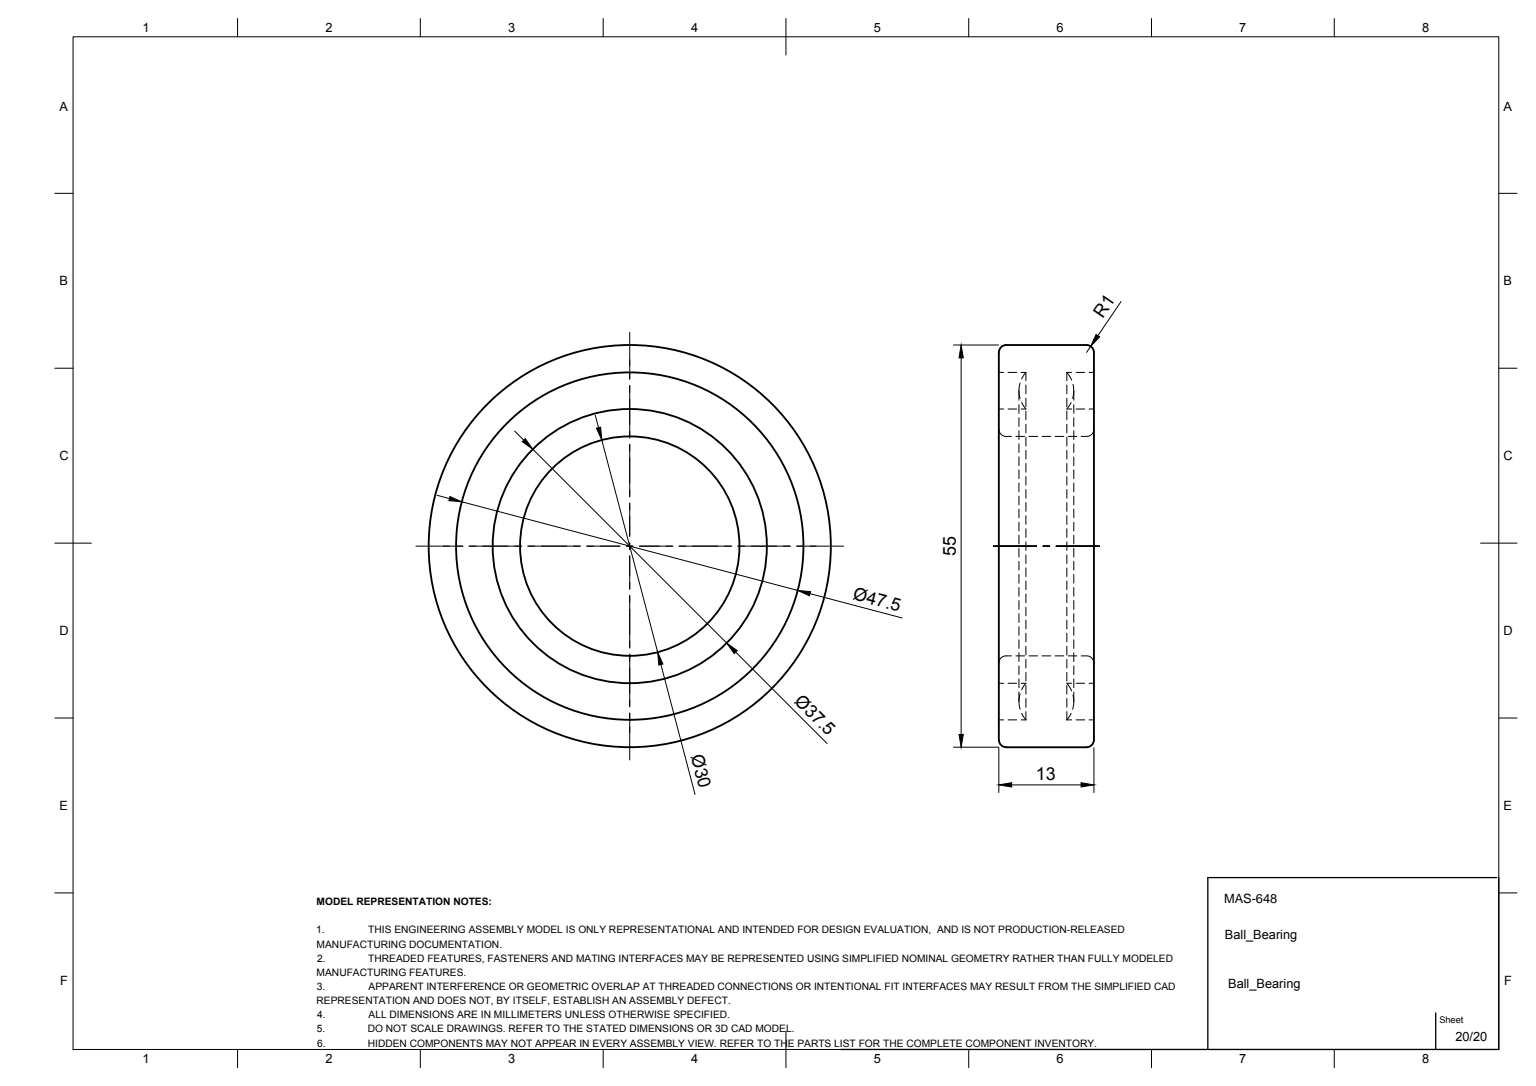
ISO-10303-21;
HEADER;
FILE_DESCRIPTION((''),'2;1');
FILE_NAME('Ball_Bearing.step','2026-10-09T12:47:58-07:00',(''),(''),'','','');
FILE_SCHEMA (('AUTOMOTIVE_DESIGN { 1 0 10303 214 3 1 1 }'));
ENDSEC;
DATA;
#10=MECHANICAL_DESIGN_GEOMETRIC_PRESENTATION_REPRESENTATION('',(#320),#3475);
#24=TOROIDAL_SURFACE('',#2119,26.5,1.) ;
#25=TOROIDAL_SURFACE('',#2125,26.5,1.) ;
#26=TOROIDAL_SURFACE('',#2136,21.25,3.75) ;
#27=TOROIDAL_SURFACE('',#2140,16.,1.) ;
#28=TOROIDAL_SURFACE('',#2146,16.,1.) ;
#29=TOROIDAL_SURFACE('',#2155,21.25,3.75) ;
#161=FACE_BOUND('',#554,.T.) ;
#162=FACE_BOUND('',#556,.T.) ;
#163=FACE_BOUND('',#558,.T.) ;
#164=FACE_BOUND('',#560,.T.) ;
#211=CIRCLE('',#2120,27.5) ;
#212=CIRCLE('',#2121,1.) ;
#213=CIRCLE('',#2122,26.5) ;
#214=CIRCLE('',#2124,27.5) ;
#215=CIRCLE('',#2126,26.5) ;
#216=CIRCLE('',#2127,1.) ;
#217=CIRCLE('',#2129,23.75) ;
#218=CIRCLE('',#2130,23.75) ;
#219=CIRCLE('',#2131,23.75) ;
#220=CIRCLE('',#2133,23.75) ;
#221=CIRCLE('',#2134,23.75) ;
#222=CIRCLE('',#2135,23.75) ;
#223=CIRCLE('',#2137,18.75) ;
#224=CIRCLE('',#2138,3.75) ;
#225=CIRCLE('',#2139,18.75) ;
#226=CIRCLE('',#2141,16.) ;
#227=CIRCLE('',#2142,1.) ;
#228=CIRCLE('',#2143,15.) ;
#229=CIRCLE('',#2145,15.) ;
#230=CIRCLE('',#2147,1.) ;
#231=CIRCLE('',#2148,16.) ;
#232=CIRCLE('',#2150,18.75) ;
#233=CIRCLE('',#2152,18.75) ;
#234=CIRCLE('',#2153,18.75) ;
#235=CIRCLE('',#2154,18.75) ;
#236=CIRCLE('',#2156,3.75) ;
#278=CYLINDRICAL_SURFACE('',#2123,27.5) ;
#279=CYLINDRICAL_SURFACE('',#2128,23.75) ;
#280=CYLINDRICAL_SURFACE('',#2132,23.75) ;
#281=CYLINDRICAL_SURFACE('',#2144,15.) ;
#282=CYLINDRICAL_SURFACE('',#2149,18.75) ;
#283=CYLINDRICAL_SURFACE('',#2151,18.75) ;
#296=SHAPE_REPRESENTATION_RELATIONSHIP('SRR','None',#3553,#308) ;
#308=ADVANCED_BREP_SHAPE_REPRESENTATION('',(#332),#3473) ;
#320=STYLED_ITEM('',(#3628),#332) ;
#332=MANIFOLD_SOLID_BREP('Body1',#1834) ;
#407=FACE_OUTER_BOUND('',#541,.T.) ;
#408=FACE_OUTER_BOUND('',#542,.T.) ;
#409=FACE_OUTER_BOUND('',#543,.T.) ;
#410=FACE_OUTER_BOUND('',#544,.T.) ;
#411=FACE_OUTER_BOUND('',#545,.T.) ;
#412=FACE_OUTER_BOUND('',#546,.T.) ;
#413=FACE_OUTER_BOUND('',#547,.T.) ;
#414=FACE_OUTER_BOUND('',#548,.T.) ;
#415=FACE_OUTER_BOUND('',#549,.T.) ;
#416=FACE_OUTER_BOUND('',#550,.T.) ;
#417=FACE_OUTER_BOUND('',#551,.T.) ;
#418=FACE_OUTER_BOUND('',#552,.T.) ;
#419=FACE_OUTER_BOUND('',#553,.T.) ;
#420=FACE_OUTER_BOUND('',#555,.T.) ;
#421=FACE_OUTER_BOUND('',#557,.T.) ;
#422=FACE_OUTER_BOUND('',#559,.T.) ;
#541=EDGE_LOOP('',(#1476,#1477,#1478,#1479)) ;
#542=EDGE_LOOP('',(#1480,#1481,#1482,#1483)) ;
#543=EDGE_LOOP('',(#1484,#1485,#1486,#1487)) ;
#544=EDGE_LOOP('',(#1488,#1489,#1490,#1491,#1492)) ;
#545=EDGE_LOOP('',(#1493,#1494,#1495,#1496,#1497)) ;
#546=EDGE_LOOP('',(#1498,#1499,#1500,#1501,#1502,#1503)) ;
#547=EDGE_LOOP('',(#1504,#1505,#1506,#1507)) ;
#548=EDGE_LOOP('',(#1508,#1509,#1510,#1511)) ;
#549=EDGE_LOOP('',(#1512,#1513,#1514,#1515)) ;
#550=EDGE_LOOP('',(#1516,#1517,#1518,#1519,#1520)) ;
#551=EDGE_LOOP('',(#1521,#1522,#1523,#1524,#1525)) ;
#552=EDGE_LOOP('',(#1526,#1527,#1528,#1529,#1530,#1531)) ;
#553=EDGE_LOOP('',(#1532)) ;
#554=EDGE_LOOP('',(#1533)) ;
#555=EDGE_LOOP('',(#1534)) ;
#556=EDGE_LOOP('',(#1535)) ;
#557=EDGE_LOOP('',(#1536)) ;
#558=EDGE_LOOP('',(#1537)) ;
#559=EDGE_LOOP('',(#1538)) ;
#560=EDGE_LOOP('',(#1539)) ;
#679=LINE('',#3241,#798) ;
#680=LINE('',#3250,#799) ;
#681=LINE('',#3260,#800) ;
#682=LINE('',#3276,#801) ;
#683=LINE('',#3284,#802) ;
#684=LINE('',#3290,#803) ;
#798=VECTOR('',#2618,27.5) ;
#799=VECTOR('',#2629,23.75) ;
#800=VECTOR('',#2640,23.75) ;
#801=VECTOR('',#2661,15.) ;
#802=VECTOR('',#2672,18.75) ;
#803=VECTOR('',#2679,18.75) ;
#919=VERTEX_POINT('',#3233) ;
#920=VERTEX_POINT('',#3235) ;
#921=VERTEX_POINT('',#3239) ;
#922=VERTEX_POINT('',#3243) ;
#923=VERTEX_POINT('',#3247) ;
#924=VERTEX_POINT('',#3249) ;
#925=VERTEX_POINT('',#3251) ;
#926=VERTEX_POINT('',#3255) ;
#927=VERTEX_POINT('',#3256) ;
#928=VERTEX_POINT('',#3259) ;
#929=VERTEX_POINT('',#3263) ;
#930=VERTEX_POINT('',#3264) ;
#931=VERTEX_POINT('',#3269) ;
#932=VERTEX_POINT('',#3271) ;
#933=VERTEX_POINT('',#3275) ;
#934=VERTEX_POINT('',#3279) ;
#935=VERTEX_POINT('',#3283) ;
#936=VERTEX_POINT('',#3287) ;
#937=VERTEX_POINT('',#3289) ;
#938=VERTEX_POINT('',#3291) ;
#1110=EDGE_CURVE('',#919,#919,#211,.T.) ;
#1111=EDGE_CURVE('',#919,#920,#212,.T.) ;
#1112=EDGE_CURVE('',#920,#920,#213,.T.) ;
#1113=EDGE_CURVE('',#921,#921,#214,.T.) ;
#1114=EDGE_CURVE('',#921,#919,#679,.T.) ;
#1115=EDGE_CURVE('',#922,#922,#215,.T.) ;
#1116=EDGE_CURVE('',#922,#921,#216,.T.) ;
#1117=EDGE_CURVE('',#923,#923,#217,.T.) ;
#1118=EDGE_CURVE('',#923,#924,#680,.T.) ;
#1119=EDGE_CURVE('',#925,#924,#218,.T.) ;
#1120=EDGE_CURVE('',#924,#925,#219,.T.) ;
#1121=EDGE_CURVE('',#926,#927,#220,.T.) ;
#1122=EDGE_CURVE('',#927,#926,#221,.T.) ;
#1123=EDGE_CURVE('',#927,#928,#681,.T.) ;
#1124=EDGE_CURVE('',#928,#928,#222,.T.) ;
#1125=EDGE_CURVE('',#929,#930,#223,.T.) ;
#1126=EDGE_CURVE('',#930,#925,#224,.T.) ;
#1127=EDGE_CURVE('',#930,#929,#225,.T.) ;
#1128=EDGE_CURVE('',#931,#931,#226,.T.) ;
#1129=EDGE_CURVE('',#931,#932,#227,.T.) ;
#1130=EDGE_CURVE('',#932,#932,#228,.T.) ;
#1131=EDGE_CURVE('',#932,#933,#682,.T.) ;
#1132=EDGE_CURVE('',#933,#933,#229,.T.) ;
#1133=EDGE_CURVE('',#933,#934,#230,.T.) ;
#1134=EDGE_CURVE('',#934,#934,#231,.T.) ;
#1135=EDGE_CURVE('',#929,#935,#683,.T.) ;
#1136=EDGE_CURVE('',#935,#935,#232,.T.) ;
#1137=EDGE_CURVE('',#936,#936,#233,.T.) ;
#1138=EDGE_CURVE('',#936,#937,#684,.T.) ;
#1139=EDGE_CURVE('',#938,#937,#234,.T.) ;
#1140=EDGE_CURVE('',#937,#938,#235,.T.) ;
#1141=EDGE_CURVE('',#926,#938,#236,.T.) ;
#1476=ORIENTED_EDGE('',*,*,#1110,.F.) ;
#1477=ORIENTED_EDGE('',*,*,#1111,.T.) ;
#1478=ORIENTED_EDGE('',*,*,#1112,.T.) ;
#1479=ORIENTED_EDGE('',*,*,#1111,.F.) ;
#1480=ORIENTED_EDGE('',*,*,#1113,.F.) ;
#1481=ORIENTED_EDGE('',*,*,#1114,.T.) ;
#1482=ORIENTED_EDGE('',*,*,#1110,.T.) ;
#1483=ORIENTED_EDGE('',*,*,#1114,.F.) ;
#1484=ORIENTED_EDGE('',*,*,#1115,.F.) ;
#1485=ORIENTED_EDGE('',*,*,#1116,.T.) ;
#1486=ORIENTED_EDGE('',*,*,#1113,.T.) ;
#1487=ORIENTED_EDGE('',*,*,#1116,.F.) ;
#1488=ORIENTED_EDGE('',*,*,#1117,.F.) ;
#1489=ORIENTED_EDGE('',*,*,#1118,.T.) ;
#1490=ORIENTED_EDGE('',*,*,#1119,.F.) ;
#1491=ORIENTED_EDGE('',*,*,#1120,.F.) ;
#1492=ORIENTED_EDGE('',*,*,#1118,.F.) ;
#1493=ORIENTED_EDGE('',*,*,#1121,.F.) ;
#1494=ORIENTED_EDGE('',*,*,#1122,.F.) ;
#1495=ORIENTED_EDGE('',*,*,#1123,.T.) ;
#1496=ORIENTED_EDGE('',*,*,#1124,.T.) ;
#1497=ORIENTED_EDGE('',*,*,#1123,.F.) ;
#1498=ORIENTED_EDGE('',*,*,#1125,.T.) ;
#1499=ORIENTED_EDGE('',*,*,#1126,.T.) ;
#1500=ORIENTED_EDGE('',*,*,#1119,.T.) ;
#1501=ORIENTED_EDGE('',*,*,#1120,.T.) ;
#1502=ORIENTED_EDGE('',*,*,#1126,.F.) ;
#1503=ORIENTED_EDGE('',*,*,#1127,.T.) ;
#1504=ORIENTED_EDGE('',*,*,#1128,.F.) ;
#1505=ORIENTED_EDGE('',*,*,#1129,.T.) ;
#1506=ORIENTED_EDGE('',*,*,#1130,.T.) ;
#1507=ORIENTED_EDGE('',*,*,#1129,.F.) ;
#1508=ORIENTED_EDGE('',*,*,#1130,.F.) ;
#1509=ORIENTED_EDGE('',*,*,#1131,.T.) ;
#1510=ORIENTED_EDGE('',*,*,#1132,.T.) ;
#1511=ORIENTED_EDGE('',*,*,#1131,.F.) ;
#1512=ORIENTED_EDGE('',*,*,#1132,.F.) ;
#1513=ORIENTED_EDGE('',*,*,#1133,.T.) ;
#1514=ORIENTED_EDGE('',*,*,#1134,.T.) ;
#1515=ORIENTED_EDGE('',*,*,#1133,.F.) ;
#1516=ORIENTED_EDGE('',*,*,#1125,.F.) ;
#1517=ORIENTED_EDGE('',*,*,#1135,.T.) ;
#1518=ORIENTED_EDGE('',*,*,#1136,.T.) ;
#1519=ORIENTED_EDGE('',*,*,#1135,.F.) ;
#1520=ORIENTED_EDGE('',*,*,#1127,.F.) ;
#1521=ORIENTED_EDGE('',*,*,#1137,.F.) ;
#1522=ORIENTED_EDGE('',*,*,#1138,.T.) ;
#1523=ORIENTED_EDGE('',*,*,#1139,.F.) ;
#1524=ORIENTED_EDGE('',*,*,#1140,.F.) ;
#1525=ORIENTED_EDGE('',*,*,#1138,.F.) ;
#1526=ORIENTED_EDGE('',*,*,#1121,.T.) ;
#1527=ORIENTED_EDGE('',*,*,#1122,.T.) ;
#1528=ORIENTED_EDGE('',*,*,#1141,.T.) ;
#1529=ORIENTED_EDGE('',*,*,#1139,.T.) ;
#1530=ORIENTED_EDGE('',*,*,#1140,.T.) ;
#1531=ORIENTED_EDGE('',*,*,#1141,.F.) ;
#1532=ORIENTED_EDGE('',*,*,#1137,.T.) ;
#1533=ORIENTED_EDGE('',*,*,#1134,.F.) ;
#1534=ORIENTED_EDGE('',*,*,#1136,.F.) ;
#1535=ORIENTED_EDGE('',*,*,#1128,.T.) ;
#1536=ORIENTED_EDGE('',*,*,#1115,.T.) ;
#1537=ORIENTED_EDGE('',*,*,#1124,.F.) ;
#1538=ORIENTED_EDGE('',*,*,#1112,.F.) ;
#1539=ORIENTED_EDGE('',*,*,#1117,.T.) ;
#1691=PLANE('',#2157) ;
#1692=PLANE('',#2158) ;
#1693=PLANE('',#2159) ;
#1694=PLANE('',#2160) ;
#1783=ADVANCED_FACE('',(#407),#24,.T.) ;
#1784=ADVANCED_FACE('',(#408),#278,.T.) ;
#1785=ADVANCED_FACE('',(#409),#25,.T.) ;
#1786=ADVANCED_FACE('',(#410),#279,.F.) ;
#1787=ADVANCED_FACE('',(#411),#280,.F.) ;
#1788=ADVANCED_FACE('',(#412),#26,.T.) ;
#1789=ADVANCED_FACE('',(#413),#27,.T.) ;
#1790=ADVANCED_FACE('',(#414),#281,.F.) ;
#1791=ADVANCED_FACE('',(#415),#28,.T.) ;
#1792=ADVANCED_FACE('',(#416),#282,.T.) ;
#1793=ADVANCED_FACE('',(#417),#283,.T.) ;
#1794=ADVANCED_FACE('',(#418),#29,.T.) ;
#1795=ADVANCED_FACE('',(#419,#161),#1691,.T.) ;
#1796=ADVANCED_FACE('',(#420,#162),#1692,.T.) ;
#1797=ADVANCED_FACE('',(#421,#163),#1693,.T.) ;
#1798=ADVANCED_FACE('',(#422,#164),#1694,.T.) ;
#1834=CLOSED_SHELL('',(#1783,#1784,#1785,#1786,#1787,#1788,#1789,#1790,
#1791,#1792,#1793,#1794,#1795,#1796,#1797,#1798)) ;
#2118=AXIS2_PLACEMENT_3D('',#3231,#2604,#2605) ;
#2119=AXIS2_PLACEMENT_3D('',#3232,#2606,#2607) ;
#2120=AXIS2_PLACEMENT_3D('',#3234,#2608,#2609) ;
#2121=AXIS2_PLACEMENT_3D('',#3236,#2610,#2611) ;
#2122=AXIS2_PLACEMENT_3D('',#3237,#2612,#2613) ;
#2123=AXIS2_PLACEMENT_3D('',#3238,#2614,#2615) ;
#2124=AXIS2_PLACEMENT_3D('',#3240,#2616,#2617) ;
#2125=AXIS2_PLACEMENT_3D('',#3242,#2619,#2620) ;
#2126=AXIS2_PLACEMENT_3D('',#3244,#2621,#2622) ;
#2127=AXIS2_PLACEMENT_3D('',#3245,#2623,#2624) ;
#2128=AXIS2_PLACEMENT_3D('',#3246,#2625,#2626) ;
#2129=AXIS2_PLACEMENT_3D('',#3248,#2627,#2628) ;
#2130=AXIS2_PLACEMENT_3D('',#3252,#2630,#2631) ;
#2131=AXIS2_PLACEMENT_3D('',#3253,#2632,#2633) ;
#2132=AXIS2_PLACEMENT_3D('',#3254,#2634,#2635) ;
#2133=AXIS2_PLACEMENT_3D('',#3257,#2636,#2637) ;
#2134=AXIS2_PLACEMENT_3D('',#3258,#2638,#2639) ;
#2135=AXIS2_PLACEMENT_3D('',#3261,#2641,#2642) ;
#2136=AXIS2_PLACEMENT_3D('',#3262,#2643,#2644) ;
#2137=AXIS2_PLACEMENT_3D('',#3265,#2645,#2646) ;
#2138=AXIS2_PLACEMENT_3D('',#3266,#2647,#2648) ;
#2139=AXIS2_PLACEMENT_3D('',#3267,#2649,#2650) ;
#2140=AXIS2_PLACEMENT_3D('',#3268,#2651,#2652) ;
#2141=AXIS2_PLACEMENT_3D('',#3270,#2653,#2654) ;
#2142=AXIS2_PLACEMENT_3D('',#3272,#2655,#2656) ;
#2143=AXIS2_PLACEMENT_3D('',#3273,#2657,#2658) ;
#2144=AXIS2_PLACEMENT_3D('',#3274,#2659,#2660) ;
#2145=AXIS2_PLACEMENT_3D('',#3277,#2662,#2663) ;
#2146=AXIS2_PLACEMENT_3D('',#3278,#2664,#2665) ;
#2147=AXIS2_PLACEMENT_3D('',#3280,#2666,#2667) ;
#2148=AXIS2_PLACEMENT_3D('',#3281,#2668,#2669) ;
#2149=AXIS2_PLACEMENT_3D('',#3282,#2670,#2671) ;
#2150=AXIS2_PLACEMENT_3D('',#3285,#2673,#2674) ;
#2151=AXIS2_PLACEMENT_3D('',#3286,#2675,#2676) ;
#2152=AXIS2_PLACEMENT_3D('',#3288,#2677,#2678) ;
#2153=AXIS2_PLACEMENT_3D('',#3292,#2680,#2681) ;
#2154=AXIS2_PLACEMENT_3D('',#3293,#2682,#2683) ;
#2155=AXIS2_PLACEMENT_3D('',#3294,#2684,#2685) ;
#2156=AXIS2_PLACEMENT_3D('',#3295,#2686,#2687) ;
#2157=AXIS2_PLACEMENT_3D('',#3296,#2688,#2689) ;
#2158=AXIS2_PLACEMENT_3D('',#3297,#2690,#2691) ;
#2159=AXIS2_PLACEMENT_3D('',#3298,#2692,#2693) ;
#2160=AXIS2_PLACEMENT_3D('',#3299,#2694,#2695) ;
#2604=DIRECTION('axis',(0.,0.,1.)) ;
#2605=DIRECTION('refdir',(1.,0.,0.)) ;
#2606=DIRECTION('center_axis',(1.,0.,0.)) ;
#2607=DIRECTION('ref_axis',(0.,0.,-1.)) ;
#2608=DIRECTION('center_axis',(1.,0.,0.)) ;
#2609=DIRECTION('ref_axis',(0.,0.,-1.)) ;
#2610=DIRECTION('center_axis',(0.,-1.,-1.22464679914735E-16)) ;
#2611=DIRECTION('ref_axis',(0.,-1.22464679914735E-16,1.)) ;
#2612=DIRECTION('center_axis',(1.,0.,0.)) ;
#2613=DIRECTION('ref_axis',(0.,0.,-1.)) ;
#2614=DIRECTION('center_axis',(1.,0.,0.)) ;
#2615=DIRECTION('ref_axis',(0.,0.,-1.)) ;
#2616=DIRECTION('center_axis',(1.,0.,0.)) ;
#2617=DIRECTION('ref_axis',(0.,0.,-1.)) ;
#2618=DIRECTION('',(-1.,0.,0.)) ;
#2619=DIRECTION('center_axis',(1.,0.,0.)) ;
#2620=DIRECTION('ref_axis',(0.,0.,-1.)) ;
#2621=DIRECTION('center_axis',(1.,0.,0.)) ;
#2622=DIRECTION('ref_axis',(0.,0.,-1.)) ;
#2623=DIRECTION('center_axis',(0.,-1.,-1.22464679914735E-16)) ;
#2624=DIRECTION('ref_axis',(0.,-1.22464679914735E-16,1.)) ;
#2625=DIRECTION('center_axis',(1.,0.,0.)) ;
#2626=DIRECTION('ref_axis',(0.,0.,-1.)) ;
#2627=DIRECTION('center_axis',(1.,0.,0.)) ;
#2628=DIRECTION('ref_axis',(0.,0.,-1.)) ;
#2629=DIRECTION('',(1.,0.,0.)) ;
#2630=DIRECTION('center_axis',(-1.,0.,0.)) ;
#2631=DIRECTION('ref_axis',(0.,0.,-1.)) ;
#2632=DIRECTION('center_axis',(-1.,0.,0.)) ;
#2633=DIRECTION('ref_axis',(0.,0.,-1.)) ;
#2634=DIRECTION('center_axis',(1.,0.,0.)) ;
#2635=DIRECTION('ref_axis',(0.,0.,-1.)) ;
#2636=DIRECTION('center_axis',(1.,0.,0.)) ;
#2637=DIRECTION('ref_axis',(0.,0.,1.)) ;
#2638=DIRECTION('center_axis',(1.,0.,0.)) ;
#2639=DIRECTION('ref_axis',(0.,0.,1.)) ;
#2640=DIRECTION('',(1.,0.,0.)) ;
#2641=DIRECTION('center_axis',(1.,0.,0.)) ;
#2642=DIRECTION('ref_axis',(0.,0.,-1.)) ;
#2643=DIRECTION('center_axis',(-1.,0.,0.)) ;
#2644=DIRECTION('ref_axis',(0.,0.,1.)) ;
#2645=DIRECTION('center_axis',(1.,0.,0.)) ;
#2646=DIRECTION('ref_axis',(0.,0.,-1.)) ;
#2647=DIRECTION('center_axis',(0.,-1.,1.22464679914735E-16)) ;
#2648=DIRECTION('ref_axis',(0.,-1.22464679914735E-16,-1.)) ;
#2649=DIRECTION('center_axis',(1.,0.,0.)) ;
#2650=DIRECTION('ref_axis',(0.,0.,-1.)) ;
#2651=DIRECTION('center_axis',(1.,0.,0.)) ;
#2652=DIRECTION('ref_axis',(0.,0.,-1.)) ;
#2653=DIRECTION('center_axis',(1.,0.,0.)) ;
#2654=DIRECTION('ref_axis',(0.,0.,-1.)) ;
#2655=DIRECTION('center_axis',(0.,-1.,-1.22464679914735E-16)) ;
#2656=DIRECTION('ref_axis',(0.,-1.22464679914735E-16,1.)) ;
#2657=DIRECTION('center_axis',(1.,0.,0.)) ;
#2658=DIRECTION('ref_axis',(0.,0.,-1.)) ;
#2659=DIRECTION('center_axis',(1.,0.,0.)) ;
#2660=DIRECTION('ref_axis',(0.,0.,-1.)) ;
#2661=DIRECTION('',(1.,0.,0.)) ;
#2662=DIRECTION('center_axis',(1.,0.,0.)) ;
#2663=DIRECTION('ref_axis',(0.,0.,-1.)) ;
#2664=DIRECTION('center_axis',(1.,0.,0.)) ;
#2665=DIRECTION('ref_axis',(0.,0.,-1.)) ;
#2666=DIRECTION('center_axis',(0.,-1.,-1.22464679914735E-16)) ;
#2667=DIRECTION('ref_axis',(0.,-1.22464679914735E-16,1.)) ;
#2668=DIRECTION('center_axis',(1.,0.,0.)) ;
#2669=DIRECTION('ref_axis',(0.,0.,-1.)) ;
#2670=DIRECTION('center_axis',(1.,0.,0.)) ;
#2671=DIRECTION('ref_axis',(0.,0.,-1.)) ;
#2672=DIRECTION('',(-1.,0.,0.)) ;
#2673=DIRECTION('center_axis',(1.,0.,0.)) ;
#2674=DIRECTION('ref_axis',(0.,0.,-1.)) ;
#2675=DIRECTION('center_axis',(1.,0.,0.)) ;
#2676=DIRECTION('ref_axis',(0.,0.,-1.)) ;
#2677=DIRECTION('center_axis',(1.,0.,0.)) ;
#2678=DIRECTION('ref_axis',(0.,0.,-1.)) ;
#2679=DIRECTION('',(-1.,0.,0.)) ;
#2680=DIRECTION('center_axis',(-1.,0.,0.)) ;
#2681=DIRECTION('ref_axis',(0.,0.,1.)) ;
#2682=DIRECTION('center_axis',(-1.,0.,0.)) ;
#2683=DIRECTION('ref_axis',(0.,0.,1.)) ;
#2684=DIRECTION('center_axis',(-1.,0.,0.)) ;
#2685=DIRECTION('ref_axis',(0.,0.,1.)) ;
#2686=DIRECTION('center_axis',(0.,-1.,1.22464679914735E-16)) ;
#2687=DIRECTION('ref_axis',(0.,-1.22464679914735E-16,-1.)) ;
#2688=DIRECTION('center_axis',(1.,0.,0.)) ;
#2689=DIRECTION('ref_axis',(0.,0.,-1.)) ;
#2690=DIRECTION('center_axis',(-1.,0.,0.)) ;
#2691=DIRECTION('ref_axis',(0.,0.,1.)) ;
#2692=DIRECTION('center_axis',(1.,0.,0.)) ;
#2693=DIRECTION('ref_axis',(0.,0.,-1.)) ;
#2694=DIRECTION('center_axis',(-1.,0.,0.)) ;
#2695=DIRECTION('ref_axis',(0.,0.,1.)) ;
#3231=CARTESIAN_POINT('',(0.,0.,0.)) ;
#3232=CARTESIAN_POINT('Origin',(-5.5,0.,0.)) ;
#3233=CARTESIAN_POINT('',(-5.5,-3.36777869765522E-15,27.5)) ;
#3234=CARTESIAN_POINT('Origin',(-5.5,0.,0.)) ;
#3235=CARTESIAN_POINT('',(-6.5,-3.24531401774049E-15,26.5)) ;
#3236=CARTESIAN_POINT('Origin',(-5.5,-3.24531401774049E-15,26.5)) ;
#3237=CARTESIAN_POINT('Origin',(-6.5,0.,0.)) ;
#3238=CARTESIAN_POINT('Origin',(-20.6375,0.,0.)) ;
#3239=CARTESIAN_POINT('',(5.5,-3.36777869765522E-15,27.5)) ;
#3240=CARTESIAN_POINT('Origin',(5.5,0.,0.)) ;
#3241=CARTESIAN_POINT('',(-20.6375,-3.36777869765522E-15,27.5)) ;
#3242=CARTESIAN_POINT('Origin',(5.5,0.,0.)) ;
#3243=CARTESIAN_POINT('',(6.5,-3.24531401774049E-15,26.5)) ;
#3244=CARTESIAN_POINT('Origin',(6.5,0.,0.)) ;
#3245=CARTESIAN_POINT('Origin',(5.5,-3.24531401774049E-15,26.5)) ;
#3246=CARTESIAN_POINT('Origin',(-20.6375,0.,0.)) ;
#3247=CARTESIAN_POINT('',(-6.5,-2.90853614797497E-15,23.75)) ;
#3248=CARTESIAN_POINT('Origin',(-6.5,0.,0.)) ;
#3249=CARTESIAN_POINT('',(-2.79508497187473,-2.90853614797496E-15,23.75)) ;
#3250=CARTESIAN_POINT('',(-20.6375,-2.90853614797496E-15,23.75)) ;
#3251=CARTESIAN_POINT('',(-2.79508497187473,2.90853614797496E-15,-23.75)) ;
#3252=CARTESIAN_POINT('Origin',(-2.79508497187473,0.,0.)) ;
#3253=CARTESIAN_POINT('Origin',(-2.79508497187473,0.,0.)) ;
#3254=CARTESIAN_POINT('Origin',(-20.6375,0.,0.)) ;
#3255=CARTESIAN_POINT('',(2.79508497187473,2.90853614797496E-15,-23.75)) ;
#3256=CARTESIAN_POINT('',(2.79508497187473,-2.90853614797496E-15,23.75)) ;
#3257=CARTESIAN_POINT('Origin',(2.79508497187473,0.,0.)) ;
#3258=CARTESIAN_POINT('Origin',(2.79508497187473,0.,0.)) ;
#3259=CARTESIAN_POINT('',(6.5,-2.90853614797497E-15,23.75)) ;
#3260=CARTESIAN_POINT('',(-20.6375,-2.90853614797496E-15,23.75)) ;
#3261=CARTESIAN_POINT('Origin',(6.5,0.,0.)) ;
#3262=CARTESIAN_POINT('Origin',(0.,0.,0.)) ;
#3263=CARTESIAN_POINT('',(-2.79508497187473,2.29621274840129E-15,18.75)) ;
#3264=CARTESIAN_POINT('',(-2.79508497187473,-2.29621274840129E-15,-18.75)) ;
#3265=CARTESIAN_POINT('Origin',(-2.79508497187473,0.,0.)) ;
#3266=CARTESIAN_POINT('Origin',(0.,-2.60237444818813E-15,-21.25)) ;
#3267=CARTESIAN_POINT('Origin',(-2.79508497187473,0.,0.)) ;
#3268=CARTESIAN_POINT('Origin',(-5.5,0.,0.)) ;
#3269=CARTESIAN_POINT('',(-6.5,-1.95943487863577E-15,16.)) ;
#3270=CARTESIAN_POINT('Origin',(-6.5,0.,0.)) ;
#3271=CARTESIAN_POINT('',(-5.5,-1.83697019872103E-15,15.)) ;
#3272=CARTESIAN_POINT('Origin',(-5.5,-1.95943487863577E-15,16.)) ;
#3273=CARTESIAN_POINT('Origin',(-5.5,0.,0.)) ;
#3274=CARTESIAN_POINT('Origin',(-20.6375,0.,0.)) ;
#3275=CARTESIAN_POINT('',(5.5,-1.83697019872103E-15,15.)) ;
#3276=CARTESIAN_POINT('',(-20.6375,-1.83697019872103E-15,15.)) ;
#3277=CARTESIAN_POINT('Origin',(5.5,0.,0.)) ;
#3278=CARTESIAN_POINT('Origin',(5.5,0.,0.)) ;
#3279=CARTESIAN_POINT('',(6.5,-1.95943487863577E-15,16.)) ;
#3280=CARTESIAN_POINT('Origin',(5.5,-1.95943487863577E-15,16.)) ;
#3281=CARTESIAN_POINT('Origin',(6.5,0.,0.)) ;
#3282=CARTESIAN_POINT('Origin',(-20.6375,0.,0.)) ;
#3283=CARTESIAN_POINT('',(-6.5,-2.29621274840129E-15,18.75)) ;
#3284=CARTESIAN_POINT('',(-20.6375,-2.29621274840129E-15,18.75)) ;
#3285=CARTESIAN_POINT('Origin',(-6.5,0.,0.)) ;
#3286=CARTESIAN_POINT('Origin',(-20.6375,0.,0.)) ;
#3287=CARTESIAN_POINT('',(6.5,-2.29621274840129E-15,18.75)) ;
#3288=CARTESIAN_POINT('Origin',(6.5,0.,0.)) ;
#3289=CARTESIAN_POINT('',(2.79508497187473,-2.29621274840129E-15,18.75)) ;
#3290=CARTESIAN_POINT('',(-20.6375,-2.29621274840129E-15,18.75)) ;
#3291=CARTESIAN_POINT('',(2.79508497187473,2.60237444818813E-15,-18.75)) ;
#3292=CARTESIAN_POINT('Origin',(2.79508497187473,0.,0.)) ;
#3293=CARTESIAN_POINT('Origin',(2.79508497187473,0.,0.)) ;
#3294=CARTESIAN_POINT('Origin',(0.,0.,0.)) ;
#3295=CARTESIAN_POINT('Origin',(0.,-2.60237444818813E-15,-21.25)) ;
#3296=CARTESIAN_POINT('Origin',(6.5,16.,0.)) ;
#3297=CARTESIAN_POINT('Origin',(-6.5,18.75,0.)) ;
#3298=CARTESIAN_POINT('Origin',(6.5,26.5,0.)) ;
#3299=CARTESIAN_POINT('Origin',(-6.5,23.75,0.)) ;
#3455=UNCERTAINTY_MEASURE_WITH_UNIT(LENGTH_MEASURE(0.01),#3476,
'DISTANCE_ACCURACY_VALUE',
'Maximum model space distance between geometric entities at asserted c
onnectivities') ;
#3457=UNCERTAINTY_MEASURE_WITH_UNIT(LENGTH_MEASURE(0.01),#3476,
'DISTANCE_ACCURACY_VALUE',
'Maximum model space distance between geometric entities at asserted c
onnectivities') ;
#3473=(
GEOMETRIC_REPRESENTATION_CONTEXT(3)
GLOBAL_UNCERTAINTY_ASSIGNED_CONTEXT((#3455))
GLOBAL_UNIT_ASSIGNED_CONTEXT((#3476,#3478,#3479))
REPRESENTATION_CONTEXT('','3D')
) ;
#3475=(
GEOMETRIC_REPRESENTATION_CONTEXT(3)
GLOBAL_UNCERTAINTY_ASSIGNED_CONTEXT((#3457))
GLOBAL_UNIT_ASSIGNED_CONTEXT((#3476,#3478,#3479))
REPRESENTATION_CONTEXT('','3D')
) ;
#3476=(
LENGTH_UNIT()
NAMED_UNIT(*)
SI_UNIT(.MILLI.,.METRE.)
) ;
#3478=(
NAMED_UNIT(*)
PLANE_ANGLE_UNIT()
SI_UNIT($,.RADIAN.)
) ;
#3479=(
NAMED_UNIT(*)
SI_UNIT($,.STERADIAN.)
SOLID_ANGLE_UNIT()
) ;
#3495=SHAPE_DEFINITION_REPRESENTATION(#3528,#3553) ;
#3528=PRODUCT_DEFINITION_SHAPE('',$,#3571) ;
#3553=SHAPE_REPRESENTATION('',(#2118),#3473) ;
#3555=PRODUCT_DEFINITION_CONTEXT('part definition',#3608,'design') ;
#3571=PRODUCT_DEFINITION('Ball_Bearing',
'Ball_Bearing',#3588,#3555) ;
#3588=PRODUCT_DEFINITION_FORMATION('',$,#3625) ;
#3608=APPLICATION_CONTEXT(
'Core Data for Automotive Mechanical Design Process') ;
#3609=PRODUCT_CONTEXT('part definition',#3608,'mechanical') ;
#3625=PRODUCT('Ball_Bearing','Ball_Bearing',
$,(#3609)) ;
#3628=PRESENTATION_STYLE_ASSIGNMENT((#3630)) ;
#3630=SURFACE_STYLE_USAGE(.BOTH.,#3632) ;
#3632=SURFACE_SIDE_STYLE('',(#3634)) ;
#3634=SURFACE_STYLE_FILL_AREA(#3636) ;
#3636=FILL_AREA_STYLE('Opaque(202,209,238)',(#3638)) ;
#3638=FILL_AREA_STYLE_COLOUR('Opaque(202,209,238)',#3640) ;
#3640=COLOUR_RGB('Opaque(202,209,238)', 0.09019608, 0.27058824, 0.51372549) ;
ENDSEC;
END-ISO-10303-21;
